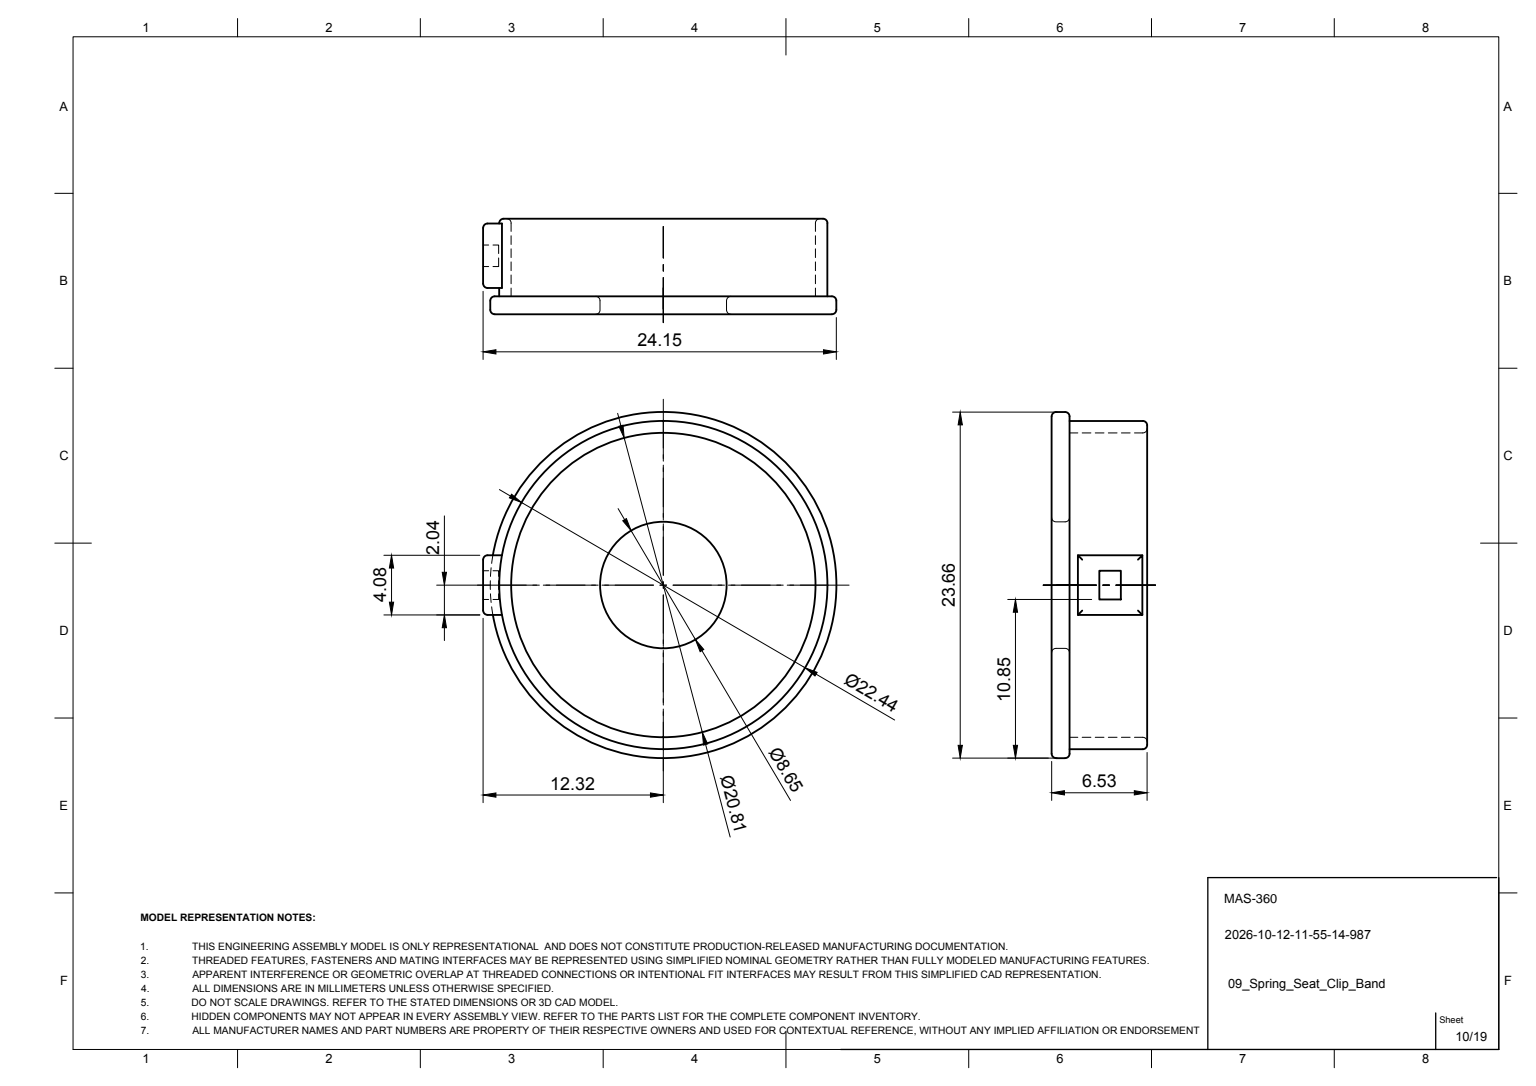
ISO-10303-21;
HEADER;
/* Generated by software containing ST-Developer
 * from STEP Tools, Inc. (www.steptools.com) 
 */

FILE_DESCRIPTION(
/* description */ (''),
/* implementation_level */ '2;1');

FILE_NAME(
/* name */ '09_Spring_Seat_Clip_Band.step',
/* time_stamp */ '2026-11-04T18:53:29-08:00',
/* author */ (''),
/* organization */ (''),
/* preprocessor_version */ 'ST-DEVELOPER v20.2',
/* originating_system */ 'Autodesk Translation Framework v15.17.0.0',
/* authorisation */ '');

FILE_SCHEMA (('AUTOMOTIVE_DESIGN { 1 0 10303 214 3 1 1 }'));
ENDSEC;

DATA;
#10=MECHANICAL_DESIGN_GEOMETRIC_PRESENTATION_REPRESENTATION('',(#1335),#100031);
#1007=CIRCLE('',#22159,4.6248);
#1008=CIRCLE('',#22160,0.3);
#1009=CIRCLE('',#22161,4.3248);
#1010=CIRCLE('',#22162,4.3248);
#1011=CIRCLE('',#22164,4.3248);
#1012=CIRCLE('',#22165,4.3248);
#1013=CIRCLE('',#22167,11.532);
#1014=CIRCLE('',#22169,0.3);
#1015=CIRCLE('',#22170,4.6248);
#1016=CIRCLE('',#22172,10.404);
#1017=CIRCLE('',#22174,10.404);
#1018=CIRCLE('',#22175,0.3);
#1019=CIRCLE('',#22176,10.704);
#1020=CIRCLE('',#22177,10.404);
#1021=CIRCLE('',#22179,10.92);
#1022=CIRCLE('',#22182,0.3);
#1023=CIRCLE('',#22183,11.22);
#1024=CIRCLE('',#22184,11.22);
#1025=CIRCLE('',#22186,11.22);
#1026=CIRCLE('',#22187,11.22);
#1027=CIRCLE('',#22188,11.22);
#1028=CIRCLE('',#22190,11.532);
#1029=CIRCLE('',#22191,0.3);
#1030=CIRCLE('',#22192,11.832);
#1031=CIRCLE('',#22193,11.832);
#1032=CIRCLE('',#22195,11.832);
#1033=CIRCLE('',#22196,11.832);
#1034=CIRCLE('',#22199,0.3);
#1276=TOROIDAL_SURFACE('',#22158,4.6248,0.3);
#1277=TOROIDAL_SURFACE('',#22168,4.6248,0.3);
#1278=TOROIDAL_SURFACE('',#22173,10.704,0.3);
#1279=TOROIDAL_SURFACE('',#22181,10.92,0.3);
#1280=TOROIDAL_SURFACE('',#22189,11.532,0.3);
#1281=TOROIDAL_SURFACE('',#22198,11.532,0.3);
#1299=SHAPE_REPRESENTATION_RELATIONSHIP('SRR','None',#100109,#1317);
#1317=ADVANCED_BREP_SHAPE_REPRESENTATION('',(#1353),#100021);
#1335=STYLED_ITEM('',(#100203),#1353);
#1353=MANIFOLD_SOLID_BREP('Body1',#20125);
#1638=PLANE('',#22166);
#1639=PLANE('',#22171);
#1640=PLANE('',#22178);
#1641=PLANE('',#22197);
#1642=PLANE('',#22208);
#1643=PLANE('',#22209);
#1644=PLANE('',#22210);
#1645=PLANE('',#22211);
#1646=PLANE('',#22212);
#1647=PLANE('',#22213);
#1648=PLANE('',#22214);
#1649=PLANE('',#22215);
#1650=PLANE('',#22216);
#1651=PLANE('',#22217);
#1776=FACE_BOUND('',#7253,.T.);
#1777=FACE_BOUND('',#7256,.T.);
#1778=FACE_BOUND('',#7259,.T.);
#1779=FACE_BOUND('',#7263,.T.);
#1780=FACE_BOUND('',#7267,.T.);
#1781=FACE_BOUND('',#7276,.T.);
#1974=ELLIPSE('',#22201,0.424264068711929,0.3);
#1975=ELLIPSE('',#22202,0.424264068711929,0.3);
#1976=ELLIPSE('',#22204,0.424264068711929,0.3);
#1977=ELLIPSE('',#22206,0.424264068711929,0.3);
#3153=LINE('',#97681,#4440);
#3154=LINE('',#97707,#4441);
#3155=LINE('',#97716,#4442);
#3156=LINE('',#97722,#4443);
#3157=LINE('',#97725,#4444);
#3158=LINE('',#97736,#4445);
#3159=LINE('',#97746,#4446);
#3160=LINE('',#97750,#4447);
#3161=LINE('',#97754,#4448);
#3162=LINE('',#97756,#4449);
#3163=LINE('',#97760,#4450);
#3164=LINE('',#97762,#4451);
#3165=LINE('',#97765,#4452);
#3166=LINE('',#97766,#4453);
#3167=LINE('',#97768,#4454);
#3168=LINE('',#97769,#4455);
#3169=LINE('',#97771,#4456);
#3170=LINE('',#97775,#4457);
#3171=LINE('',#97777,#4458);
#3172=LINE('',#97779,#4459);
#3173=LINE('',#97780,#4460);
#3174=LINE('',#97783,#4461);
#3175=LINE('',#97785,#4462);
#3176=LINE('',#97786,#4463);
#3177=LINE('',#97789,#4464);
#3178=LINE('',#97790,#4465);
#3179=LINE('',#97793,#4466);
#3180=LINE('',#97794,#4467);
#3181=LINE('',#97796,#4468);
#3182=LINE('',#97799,#4469);
#4440=VECTOR('',#27358,4.3248);
#4441=VECTOR('',#27393,10.404);
#4442=VECTOR('',#27404,11.22);
#4443=VECTOR('',#27409,10.);
#4444=VECTOR('',#27412,10.);
#4445=VECTOR('',#27425,11.832);
#4446=VECTOR('',#27438,10.);
#4447=VECTOR('',#27441,10.);
#4448=VECTOR('',#27446,10.);
#4449=VECTOR('',#27447,10.);
#4450=VECTOR('',#27452,10.);
#4451=VECTOR('',#27453,10.);
#4452=VECTOR('',#27458,10.);
#4453=VECTOR('',#27459,10.);
#4454=VECTOR('',#27462,10.);
#4455=VECTOR('',#27463,10.);
#4456=VECTOR('',#27466,10.);
#4457=VECTOR('',#27469,10.);
#4458=VECTOR('',#27470,10.);
#4459=VECTOR('',#27471,10.);
#4460=VECTOR('',#27472,10.);
#4461=VECTOR('',#27475,10.);
#4462=VECTOR('',#27476,10.);
#4463=VECTOR('',#27477,10.);
#4464=VECTOR('',#27480,10.);
#4465=VECTOR('',#27481,10.);
#4466=VECTOR('',#27484,10.);
#4467=VECTOR('',#27485,10.);
#4468=VECTOR('',#27488,10.);
#4469=VECTOR('',#27493,10.);
#4972=CYLINDRICAL_SURFACE('',#22163,4.3248);
#4973=CYLINDRICAL_SURFACE('',#22180,10.404);
#4974=CYLINDRICAL_SURFACE('',#22185,11.22);
#4975=CYLINDRICAL_SURFACE('',#22194,11.832);
#4976=CYLINDRICAL_SURFACE('',#22200,0.3);
#4977=CYLINDRICAL_SURFACE('',#22203,0.3);
#4978=CYLINDRICAL_SURFACE('',#22205,0.3);
#4979=CYLINDRICAL_SURFACE('',#22207,0.3);
#6011=FACE_OUTER_BOUND('',#7250,.T.);
#6012=FACE_OUTER_BOUND('',#7251,.T.);
#6013=FACE_OUTER_BOUND('',#7252,.T.);
#6014=FACE_OUTER_BOUND('',#7254,.T.);
#6015=FACE_OUTER_BOUND('',#7255,.T.);
#6016=FACE_OUTER_BOUND('',#7257,.T.);
#6017=FACE_OUTER_BOUND('',#7258,.T.);
#6018=FACE_OUTER_BOUND('',#7260,.T.);
#6019=FACE_OUTER_BOUND('',#7261,.T.);
#6020=FACE_OUTER_BOUND('',#7262,.T.);
#6021=FACE_OUTER_BOUND('',#7264,.T.);
#6022=FACE_OUTER_BOUND('',#7265,.T.);
#6023=FACE_OUTER_BOUND('',#7266,.T.);
#6024=FACE_OUTER_BOUND('',#7268,.T.);
#6025=FACE_OUTER_BOUND('',#7269,.T.);
#6026=FACE_OUTER_BOUND('',#7270,.T.);
#6027=FACE_OUTER_BOUND('',#7271,.T.);
#6028=FACE_OUTER_BOUND('',#7272,.T.);
#6029=FACE_OUTER_BOUND('',#7273,.T.);
#6030=FACE_OUTER_BOUND('',#7274,.T.);
#6031=FACE_OUTER_BOUND('',#7275,.T.);
#6032=FACE_OUTER_BOUND('',#7277,.T.);
#6033=FACE_OUTER_BOUND('',#7278,.T.);
#6034=FACE_OUTER_BOUND('',#7279,.T.);
#6035=FACE_OUTER_BOUND('',#7280,.T.);
#6036=FACE_OUTER_BOUND('',#7281,.T.);
#6037=FACE_OUTER_BOUND('',#7282,.T.);
#6038=FACE_OUTER_BOUND('',#7283,.T.);
#7250=EDGE_LOOP('',(#18177,#18178,#18179,#18180,#18181));
#7251=EDGE_LOOP('',(#18182,#18183,#18184,#18185,#18186,#18187));
#7252=EDGE_LOOP('',(#18188));
#7253=EDGE_LOOP('',(#18189));
#7254=EDGE_LOOP('',(#18190,#18191,#18192,#18193,#18194));
#7255=EDGE_LOOP('',(#18195));
#7256=EDGE_LOOP('',(#18196));
#7257=EDGE_LOOP('',(#18197,#18198,#18199,#18200,#18201));
#7258=EDGE_LOOP('',(#18202));
#7259=EDGE_LOOP('',(#18203));
#7260=EDGE_LOOP('',(#18204,#18205,#18206,#18207,#18208));
#7261=EDGE_LOOP('',(#18209,#18210,#18211,#18212,#18213));
#7262=EDGE_LOOP('',(#18214,#18215,#18216,#18217,#18218));
#7263=EDGE_LOOP('',(#18219,#18220,#18221,#18222));
#7264=EDGE_LOOP('',(#18223,#18224,#18225,#18226,#18227));
#7265=EDGE_LOOP('',(#18228,#18229,#18230,#18231,#18232,#18233));
#7266=EDGE_LOOP('',(#18234));
#7267=EDGE_LOOP('',(#18235));
#7268=EDGE_LOOP('',(#18236,#18237,#18238,#18239,#18240));
#7269=EDGE_LOOP('',(#18241,#18242,#18243,#18244));
#7270=EDGE_LOOP('',(#18245,#18246,#18247,#18248));
#7271=EDGE_LOOP('',(#18249,#18250,#18251,#18252));
#7272=EDGE_LOOP('',(#18253,#18254,#18255,#18256));
#7273=EDGE_LOOP('',(#18257,#18258,#18259,#18260));
#7274=EDGE_LOOP('',(#18261,#18262,#18263,#18264));
#7275=EDGE_LOOP('',(#18265,#18266,#18267,#18268));
#7276=EDGE_LOOP('',(#18269,#18270,#18271,#18272));
#7277=EDGE_LOOP('',(#18273,#18274,#18275,#18276));
#7278=EDGE_LOOP('',(#18277,#18278,#18279,#18280));
#7279=EDGE_LOOP('',(#18281,#18282,#18283,#18284));
#7280=EDGE_LOOP('',(#18285,#18286,#18287,#18288));
#7281=EDGE_LOOP('',(#18289,#18290,#18291,#18292));
#7282=EDGE_LOOP('',(#18293,#18294,#18295,#18296));
#7283=EDGE_LOOP('',(#18297,#18298,#18299,#18300));
#9719=VERTEX_POINT('',#97672);
#9720=VERTEX_POINT('',#97674);
#9721=VERTEX_POINT('',#97676);
#9722=VERTEX_POINT('',#97680);
#9723=VERTEX_POINT('',#97682);
#9724=VERTEX_POINT('',#97686);
#9725=VERTEX_POINT('',#97689);
#9726=VERTEX_POINT('',#97693);
#9727=VERTEX_POINT('',#97696);
#9728=VERTEX_POINT('',#97697);
#9729=VERTEX_POINT('',#97699);
#9730=VERTEX_POINT('',#97704);
#9731=VERTEX_POINT('',#97709);
#9732=VERTEX_POINT('',#97711);
#9733=VERTEX_POINT('',#97715);
#9734=VERTEX_POINT('',#97718);
#9735=VERTEX_POINT('',#97719);
#9736=VERTEX_POINT('',#97721);
#9737=VERTEX_POINT('',#97723);
#9738=VERTEX_POINT('',#97727);
#9739=VERTEX_POINT('',#97729);
#9740=VERTEX_POINT('',#97731);
#9741=VERTEX_POINT('',#97735);
#9742=VERTEX_POINT('',#97737);
#9743=VERTEX_POINT('',#97744);
#9744=VERTEX_POINT('',#97745);
#9745=VERTEX_POINT('',#97747);
#9746=VERTEX_POINT('',#97749);
#9747=VERTEX_POINT('',#97753);
#9748=VERTEX_POINT('',#97755);
#9749=VERTEX_POINT('',#97759);
#9750=VERTEX_POINT('',#97761);
#9751=VERTEX_POINT('',#97773);
#9752=VERTEX_POINT('',#97774);
#9753=VERTEX_POINT('',#97776);
#9754=VERTEX_POINT('',#97778);
#9755=VERTEX_POINT('',#97782);
#9756=VERTEX_POINT('',#97784);
#9757=VERTEX_POINT('',#97788);
#9758=VERTEX_POINT('',#97792);
#12563=EDGE_CURVE('',#9719,#9719,#1007,.T.);
#12564=EDGE_CURVE('',#9719,#9720,#1008,.T.);
#12565=EDGE_CURVE('',#9720,#9721,#1009,.T.);
#12566=EDGE_CURVE('',#9721,#9720,#1010,.T.);
#12567=EDGE_CURVE('',#9721,#9722,#3153,.T.);
#12568=EDGE_CURVE('',#9723,#9722,#1011,.T.);
#12569=EDGE_CURVE('',#9722,#9723,#1012,.T.);
#12570=EDGE_CURVE('',#9724,#9724,#1013,.T.);
#12571=EDGE_CURVE('',#9723,#9725,#1014,.T.);
#12572=EDGE_CURVE('',#9725,#9725,#1015,.T.);
#12573=EDGE_CURVE('',#9726,#9726,#1016,.T.);
#12574=EDGE_CURVE('',#9727,#9728,#1017,.T.);
#12575=EDGE_CURVE('',#9728,#9729,#1018,.T.);
#12576=EDGE_CURVE('',#9729,#9729,#1019,.T.);
#12577=EDGE_CURVE('',#9728,#9727,#1020,.T.);
#12578=EDGE_CURVE('',#9730,#9730,#1021,.T.);
#12579=EDGE_CURVE('',#9726,#9727,#3154,.T.);
#12580=EDGE_CURVE('',#9730,#9731,#1022,.T.);
#12581=EDGE_CURVE('',#9731,#9732,#1023,.T.);
#12582=EDGE_CURVE('',#9732,#9731,#1024,.T.);
#12583=EDGE_CURVE('',#9732,#9733,#3155,.T.);
#12584=EDGE_CURVE('',#9733,#9733,#1025,.T.);
#12585=EDGE_CURVE('',#9734,#9735,#1026,.T.);
#12586=EDGE_CURVE('',#9735,#9736,#3156,.T.);
#12587=EDGE_CURVE('',#9736,#9737,#1027,.T.);
#12588=EDGE_CURVE('',#9737,#9734,#3157,.T.);
#12589=EDGE_CURVE('',#9738,#9738,#1028,.T.);
#12590=EDGE_CURVE('',#9738,#9739,#1029,.T.);
#12591=EDGE_CURVE('',#9739,#9740,#1030,.T.);
#12592=EDGE_CURVE('',#9740,#9739,#1031,.T.);
#12593=EDGE_CURVE('',#9740,#9741,#3158,.T.);
#12594=EDGE_CURVE('',#9742,#9741,#1032,.T.);
#12595=EDGE_CURVE('',#9741,#9742,#1033,.T.);
#12596=EDGE_CURVE('',#9742,#9724,#1034,.T.);
#12597=EDGE_CURVE('',#9743,#9744,#3159,.T.);
#12598=EDGE_CURVE('',#9744,#9745,#1974,.T.);
#12599=EDGE_CURVE('',#9745,#9746,#3160,.T.);
#12600=EDGE_CURVE('',#9746,#9743,#1975,.T.);
#12601=EDGE_CURVE('',#9747,#9745,#3161,.T.);
#12602=EDGE_CURVE('',#9744,#9748,#3162,.T.);
#12603=EDGE_CURVE('',#9748,#9747,#1976,.T.);
#12604=EDGE_CURVE('',#9749,#9743,#3163,.T.);
#12605=EDGE_CURVE('',#9746,#9750,#3164,.T.);
#12606=EDGE_CURVE('',#9750,#9749,#1977,.T.);
#12607=EDGE_CURVE('',#9748,#9749,#3165,.T.);
#12608=EDGE_CURVE('',#9750,#9747,#3166,.T.);
#12609=EDGE_CURVE('',#9735,#9744,#3167,.T.);
#12610=EDGE_CURVE('',#9748,#9734,#3168,.T.);
#12611=EDGE_CURVE('',#9743,#9736,#3169,.T.);
#12612=EDGE_CURVE('',#9751,#9752,#3170,.T.);
#12613=EDGE_CURVE('',#9752,#9753,#3171,.T.);
#12614=EDGE_CURVE('',#9753,#9754,#3172,.T.);
#12615=EDGE_CURVE('',#9754,#9751,#3173,.T.);
#12616=EDGE_CURVE('',#9751,#9755,#3174,.T.);
#12617=EDGE_CURVE('',#9755,#9756,#3175,.T.);
#12618=EDGE_CURVE('',#9752,#9756,#3176,.T.);
#12619=EDGE_CURVE('',#9754,#9757,#3177,.T.);
#12620=EDGE_CURVE('',#9757,#9755,#3178,.T.);
#12621=EDGE_CURVE('',#9753,#9758,#3179,.T.);
#12622=EDGE_CURVE('',#9758,#9757,#3180,.T.);
#12623=EDGE_CURVE('',#9756,#9758,#3181,.T.);
#12624=EDGE_CURVE('',#9737,#9749,#3182,.T.);
#18177=ORIENTED_EDGE('',*,*,#12563,.T.);
#18178=ORIENTED_EDGE('',*,*,#12564,.T.);
#18179=ORIENTED_EDGE('',*,*,#12565,.T.);
#18180=ORIENTED_EDGE('',*,*,#12566,.T.);
#18181=ORIENTED_EDGE('',*,*,#12564,.F.);
#18182=ORIENTED_EDGE('',*,*,#12566,.F.);
#18183=ORIENTED_EDGE('',*,*,#12567,.T.);
#18184=ORIENTED_EDGE('',*,*,#12568,.F.);
#18185=ORIENTED_EDGE('',*,*,#12569,.F.);
#18186=ORIENTED_EDGE('',*,*,#12567,.F.);
#18187=ORIENTED_EDGE('',*,*,#12565,.F.);
#18188=ORIENTED_EDGE('',*,*,#12570,.F.);
#18189=ORIENTED_EDGE('',*,*,#12563,.F.);
#18190=ORIENTED_EDGE('',*,*,#12568,.T.);
#18191=ORIENTED_EDGE('',*,*,#12569,.T.);
#18192=ORIENTED_EDGE('',*,*,#12571,.T.);
#18193=ORIENTED_EDGE('',*,*,#12572,.T.);
#18194=ORIENTED_EDGE('',*,*,#12571,.F.);
#18195=ORIENTED_EDGE('',*,*,#12573,.T.);
#18196=ORIENTED_EDGE('',*,*,#12572,.F.);
#18197=ORIENTED_EDGE('',*,*,#12574,.T.);
#18198=ORIENTED_EDGE('',*,*,#12575,.T.);
#18199=ORIENTED_EDGE('',*,*,#12576,.T.);
#18200=ORIENTED_EDGE('',*,*,#12575,.F.);
#18201=ORIENTED_EDGE('',*,*,#12577,.T.);
#18202=ORIENTED_EDGE('',*,*,#12578,.F.);
#18203=ORIENTED_EDGE('',*,*,#12576,.F.);
#18204=ORIENTED_EDGE('',*,*,#12573,.F.);
#18205=ORIENTED_EDGE('',*,*,#12579,.T.);
#18206=ORIENTED_EDGE('',*,*,#12577,.F.);
#18207=ORIENTED_EDGE('',*,*,#12574,.F.);
#18208=ORIENTED_EDGE('',*,*,#12579,.F.);
#18209=ORIENTED_EDGE('',*,*,#12578,.T.);
#18210=ORIENTED_EDGE('',*,*,#12580,.T.);
#18211=ORIENTED_EDGE('',*,*,#12581,.T.);
#18212=ORIENTED_EDGE('',*,*,#12582,.T.);
#18213=ORIENTED_EDGE('',*,*,#12580,.F.);
#18214=ORIENTED_EDGE('',*,*,#12582,.F.);
#18215=ORIENTED_EDGE('',*,*,#12583,.T.);
#18216=ORIENTED_EDGE('',*,*,#12584,.T.);
#18217=ORIENTED_EDGE('',*,*,#12583,.F.);
#18218=ORIENTED_EDGE('',*,*,#12581,.F.);
#18219=ORIENTED_EDGE('',*,*,#12585,.T.);
#18220=ORIENTED_EDGE('',*,*,#12586,.T.);
#18221=ORIENTED_EDGE('',*,*,#12587,.T.);
#18222=ORIENTED_EDGE('',*,*,#12588,.T.);
#18223=ORIENTED_EDGE('',*,*,#12589,.T.);
#18224=ORIENTED_EDGE('',*,*,#12590,.T.);
#18225=ORIENTED_EDGE('',*,*,#12591,.T.);
#18226=ORIENTED_EDGE('',*,*,#12592,.T.);
#18227=ORIENTED_EDGE('',*,*,#12590,.F.);
#18228=ORIENTED_EDGE('',*,*,#12592,.F.);
#18229=ORIENTED_EDGE('',*,*,#12593,.T.);
#18230=ORIENTED_EDGE('',*,*,#12594,.F.);
#18231=ORIENTED_EDGE('',*,*,#12595,.F.);
#18232=ORIENTED_EDGE('',*,*,#12593,.F.);
#18233=ORIENTED_EDGE('',*,*,#12591,.F.);
#18234=ORIENTED_EDGE('',*,*,#12589,.F.);
#18235=ORIENTED_EDGE('',*,*,#12584,.F.);
#18236=ORIENTED_EDGE('',*,*,#12594,.T.);
#18237=ORIENTED_EDGE('',*,*,#12595,.T.);
#18238=ORIENTED_EDGE('',*,*,#12596,.T.);
#18239=ORIENTED_EDGE('',*,*,#12570,.T.);
#18240=ORIENTED_EDGE('',*,*,#12596,.F.);
#18241=ORIENTED_EDGE('',*,*,#12597,.T.);
#18242=ORIENTED_EDGE('',*,*,#12598,.T.);
#18243=ORIENTED_EDGE('',*,*,#12599,.T.);
#18244=ORIENTED_EDGE('',*,*,#12600,.T.);
#18245=ORIENTED_EDGE('',*,*,#12601,.T.);
#18246=ORIENTED_EDGE('',*,*,#12598,.F.);
#18247=ORIENTED_EDGE('',*,*,#12602,.T.);
#18248=ORIENTED_EDGE('',*,*,#12603,.T.);
#18249=ORIENTED_EDGE('',*,*,#12604,.T.);
#18250=ORIENTED_EDGE('',*,*,#12600,.F.);
#18251=ORIENTED_EDGE('',*,*,#12605,.T.);
#18252=ORIENTED_EDGE('',*,*,#12606,.T.);
#18253=ORIENTED_EDGE('',*,*,#12607,.T.);
#18254=ORIENTED_EDGE('',*,*,#12606,.F.);
#18255=ORIENTED_EDGE('',*,*,#12608,.T.);
#18256=ORIENTED_EDGE('',*,*,#12603,.F.);
#18257=ORIENTED_EDGE('',*,*,#12602,.F.);
#18258=ORIENTED_EDGE('',*,*,#12609,.F.);
#18259=ORIENTED_EDGE('',*,*,#12585,.F.);
#18260=ORIENTED_EDGE('',*,*,#12610,.F.);
#18261=ORIENTED_EDGE('',*,*,#12597,.F.);
#18262=ORIENTED_EDGE('',*,*,#12611,.T.);
#18263=ORIENTED_EDGE('',*,*,#12586,.F.);
#18264=ORIENTED_EDGE('',*,*,#12609,.T.);
#18265=ORIENTED_EDGE('',*,*,#12599,.F.);
#18266=ORIENTED_EDGE('',*,*,#12601,.F.);
#18267=ORIENTED_EDGE('',*,*,#12608,.F.);
#18268=ORIENTED_EDGE('',*,*,#12605,.F.);
#18269=ORIENTED_EDGE('',*,*,#12612,.T.);
#18270=ORIENTED_EDGE('',*,*,#12613,.T.);
#18271=ORIENTED_EDGE('',*,*,#12614,.T.);
#18272=ORIENTED_EDGE('',*,*,#12615,.T.);
#18273=ORIENTED_EDGE('',*,*,#12612,.F.);
#18274=ORIENTED_EDGE('',*,*,#12616,.T.);
#18275=ORIENTED_EDGE('',*,*,#12617,.T.);
#18276=ORIENTED_EDGE('',*,*,#12618,.F.);
#18277=ORIENTED_EDGE('',*,*,#12615,.F.);
#18278=ORIENTED_EDGE('',*,*,#12619,.T.);
#18279=ORIENTED_EDGE('',*,*,#12620,.T.);
#18280=ORIENTED_EDGE('',*,*,#12616,.F.);
#18281=ORIENTED_EDGE('',*,*,#12614,.F.);
#18282=ORIENTED_EDGE('',*,*,#12621,.T.);
#18283=ORIENTED_EDGE('',*,*,#12622,.T.);
#18284=ORIENTED_EDGE('',*,*,#12619,.F.);
#18285=ORIENTED_EDGE('',*,*,#12613,.F.);
#18286=ORIENTED_EDGE('',*,*,#12618,.T.);
#18287=ORIENTED_EDGE('',*,*,#12623,.T.);
#18288=ORIENTED_EDGE('',*,*,#12621,.F.);
#18289=ORIENTED_EDGE('',*,*,#12623,.F.);
#18290=ORIENTED_EDGE('',*,*,#12617,.F.);
#18291=ORIENTED_EDGE('',*,*,#12620,.F.);
#18292=ORIENTED_EDGE('',*,*,#12622,.F.);
#18293=ORIENTED_EDGE('',*,*,#12604,.F.);
#18294=ORIENTED_EDGE('',*,*,#12624,.F.);
#18295=ORIENTED_EDGE('',*,*,#12587,.F.);
#18296=ORIENTED_EDGE('',*,*,#12611,.F.);
#18297=ORIENTED_EDGE('',*,*,#12607,.F.);
#18298=ORIENTED_EDGE('',*,*,#12610,.T.);
#18299=ORIENTED_EDGE('',*,*,#12588,.F.);
#18300=ORIENTED_EDGE('',*,*,#12624,.T.);
#19945=ADVANCED_FACE('',(#6011),#1276,.T.);
#19946=ADVANCED_FACE('',(#6012),#4972,.F.);
#19947=ADVANCED_FACE('',(#6013,#1776),#1638,.T.);
#19948=ADVANCED_FACE('',(#6014),#1277,.T.);
#19949=ADVANCED_FACE('',(#6015,#1777),#1639,.T.);
#19950=ADVANCED_FACE('',(#6016),#1278,.T.);
#19951=ADVANCED_FACE('',(#6017,#1778),#1640,.T.);
#19952=ADVANCED_FACE('',(#6018),#4973,.F.);
#19953=ADVANCED_FACE('',(#6019),#1279,.T.);
#19954=ADVANCED_FACE('',(#6020,#1779),#4974,.T.);
#19955=ADVANCED_FACE('',(#6021),#1280,.T.);
#19956=ADVANCED_FACE('',(#6022),#4975,.T.);
#19957=ADVANCED_FACE('',(#6023,#1780),#1641,.T.);
#19958=ADVANCED_FACE('',(#6024),#1281,.T.);
#19959=ADVANCED_FACE('',(#6025),#4976,.T.);
#19960=ADVANCED_FACE('',(#6026),#4977,.T.);
#19961=ADVANCED_FACE('',(#6027),#4978,.T.);
#19962=ADVANCED_FACE('',(#6028),#4979,.T.);
#19963=ADVANCED_FACE('',(#6029),#1642,.T.);
#19964=ADVANCED_FACE('',(#6030),#1643,.F.);
#19965=ADVANCED_FACE('',(#6031,#1781),#1644,.T.);
#19966=ADVANCED_FACE('',(#6032),#1645,.F.);
#19967=ADVANCED_FACE('',(#6033),#1646,.F.);
#19968=ADVANCED_FACE('',(#6034),#1647,.F.);
#19969=ADVANCED_FACE('',(#6035),#1648,.F.);
#19970=ADVANCED_FACE('',(#6036),#1649,.F.);
#19971=ADVANCED_FACE('',(#6037),#1650,.T.);
#19972=ADVANCED_FACE('',(#6038),#1651,.T.);
#20125=CLOSED_SHELL('',(#19945,#19946,#19947,#19948,#19949,#19950,#19951,
#19952,#19953,#19954,#19955,#19956,#19957,#19958,#19959,#19960,#19961,#19962,
#19963,#19964,#19965,#19966,#19967,#19968,#19969,#19970,#19971,#19972));
#22157=AXIS2_PLACEMENT_3D('',#97670,#27344,#27345);
#22158=AXIS2_PLACEMENT_3D('',#97671,#27346,#27347);
#22159=AXIS2_PLACEMENT_3D('',#97673,#27348,#27349);
#22160=AXIS2_PLACEMENT_3D('',#97675,#27350,#27351);
#22161=AXIS2_PLACEMENT_3D('',#97677,#27352,#27353);
#22162=AXIS2_PLACEMENT_3D('',#97678,#27354,#27355);
#22163=AXIS2_PLACEMENT_3D('',#97679,#27356,#27357);
#22164=AXIS2_PLACEMENT_3D('',#97683,#27359,#27360);
#22165=AXIS2_PLACEMENT_3D('',#97684,#27361,#27362);
#22166=AXIS2_PLACEMENT_3D('',#97685,#27363,#27364);
#22167=AXIS2_PLACEMENT_3D('',#97687,#27365,#27366);
#22168=AXIS2_PLACEMENT_3D('',#97688,#27367,#27368);
#22169=AXIS2_PLACEMENT_3D('',#97690,#27369,#27370);
#22170=AXIS2_PLACEMENT_3D('',#97691,#27371,#27372);
#22171=AXIS2_PLACEMENT_3D('',#97692,#27373,#27374);
#22172=AXIS2_PLACEMENT_3D('',#97694,#27375,#27376);
#22173=AXIS2_PLACEMENT_3D('',#97695,#27377,#27378);
#22174=AXIS2_PLACEMENT_3D('',#97698,#27379,#27380);
#22175=AXIS2_PLACEMENT_3D('',#97700,#27381,#27382);
#22176=AXIS2_PLACEMENT_3D('',#97701,#27383,#27384);
#22177=AXIS2_PLACEMENT_3D('',#97702,#27385,#27386);
#22178=AXIS2_PLACEMENT_3D('',#97703,#27387,#27388);
#22179=AXIS2_PLACEMENT_3D('',#97705,#27389,#27390);
#22180=AXIS2_PLACEMENT_3D('',#97706,#27391,#27392);
#22181=AXIS2_PLACEMENT_3D('',#97708,#27394,#27395);
#22182=AXIS2_PLACEMENT_3D('',#97710,#27396,#27397);
#22183=AXIS2_PLACEMENT_3D('',#97712,#27398,#27399);
#22184=AXIS2_PLACEMENT_3D('',#97713,#27400,#27401);
#22185=AXIS2_PLACEMENT_3D('',#97714,#27402,#27403);
#22186=AXIS2_PLACEMENT_3D('',#97717,#27405,#27406);
#22187=AXIS2_PLACEMENT_3D('',#97720,#27407,#27408);
#22188=AXIS2_PLACEMENT_3D('',#97724,#27410,#27411);
#22189=AXIS2_PLACEMENT_3D('',#97726,#27413,#27414);
#22190=AXIS2_PLACEMENT_3D('',#97728,#27415,#27416);
#22191=AXIS2_PLACEMENT_3D('',#97730,#27417,#27418);
#22192=AXIS2_PLACEMENT_3D('',#97732,#27419,#27420);
#22193=AXIS2_PLACEMENT_3D('',#97733,#27421,#27422);
#22194=AXIS2_PLACEMENT_3D('',#97734,#27423,#27424);
#22195=AXIS2_PLACEMENT_3D('',#97738,#27426,#27427);
#22196=AXIS2_PLACEMENT_3D('',#97739,#27428,#27429);
#22197=AXIS2_PLACEMENT_3D('',#97740,#27430,#27431);
#22198=AXIS2_PLACEMENT_3D('',#97741,#27432,#27433);
#22199=AXIS2_PLACEMENT_3D('',#97742,#27434,#27435);
#22200=AXIS2_PLACEMENT_3D('',#97743,#27436,#27437);
#22201=AXIS2_PLACEMENT_3D('',#97748,#27439,#27440);
#22202=AXIS2_PLACEMENT_3D('',#97751,#27442,#27443);
#22203=AXIS2_PLACEMENT_3D('',#97752,#27444,#27445);
#22204=AXIS2_PLACEMENT_3D('',#97757,#27448,#27449);
#22205=AXIS2_PLACEMENT_3D('',#97758,#27450,#27451);
#22206=AXIS2_PLACEMENT_3D('',#97763,#27454,#27455);
#22207=AXIS2_PLACEMENT_3D('',#97764,#27456,#27457);
#22208=AXIS2_PLACEMENT_3D('',#97767,#27460,#27461);
#22209=AXIS2_PLACEMENT_3D('',#97770,#27464,#27465);
#22210=AXIS2_PLACEMENT_3D('',#97772,#27467,#27468);
#22211=AXIS2_PLACEMENT_3D('',#97781,#27473,#27474);
#22212=AXIS2_PLACEMENT_3D('',#97787,#27478,#27479);
#22213=AXIS2_PLACEMENT_3D('',#97791,#27482,#27483);
#22214=AXIS2_PLACEMENT_3D('',#97795,#27486,#27487);
#22215=AXIS2_PLACEMENT_3D('',#97797,#27489,#27490);
#22216=AXIS2_PLACEMENT_3D('',#97798,#27491,#27492);
#22217=AXIS2_PLACEMENT_3D('',#97800,#27494,#27495);
#27344=DIRECTION('axis',(0.,0.,1.));
#27345=DIRECTION('refdir',(1.,0.,0.));
#27346=DIRECTION('center_axis',(1.,0.,0.));
#27347=DIRECTION('ref_axis',(0.,0.,-1.));
#27348=DIRECTION('center_axis',(-1.,0.,0.));
#27349=DIRECTION('ref_axis',(0.,-1.,1.83697019872103E-16));
#27350=DIRECTION('center_axis',(0.,-1.,-1.22464679914735E-16));
#27351=DIRECTION('ref_axis',(0.,-1.22464679914735E-16,1.));
#27352=DIRECTION('center_axis',(1.,0.,0.));
#27353=DIRECTION('ref_axis',(0.,-1.,1.83697019872103E-16));
#27354=DIRECTION('center_axis',(1.,0.,0.));
#27355=DIRECTION('ref_axis',(0.,-1.,1.83697019872103E-16));
#27356=DIRECTION('center_axis',(1.,0.,0.));
#27357=DIRECTION('ref_axis',(0.,1.,0.));
#27358=DIRECTION('',(1.,0.,0.));
#27359=DIRECTION('center_axis',(-1.,0.,0.));
#27360=DIRECTION('ref_axis',(0.,-1.,1.83697019872103E-16));
#27361=DIRECTION('center_axis',(-1.,0.,0.));
#27362=DIRECTION('ref_axis',(0.,-1.,1.83697019872103E-16));
#27363=DIRECTION('center_axis',(-1.,0.,0.));
#27364=DIRECTION('ref_axis',(0.,0.,1.));
#27365=DIRECTION('center_axis',(1.,0.,0.));
#27366=DIRECTION('ref_axis',(0.,-1.,1.83697019872103E-16));
#27367=DIRECTION('center_axis',(1.,0.,0.));
#27368=DIRECTION('ref_axis',(0.,0.,-1.));
#27369=DIRECTION('center_axis',(0.,-1.,-1.22464679914735E-16));
#27370=DIRECTION('ref_axis',(0.,-1.22464679914735E-16,1.));
#27371=DIRECTION('center_axis',(1.,0.,0.));
#27372=DIRECTION('ref_axis',(0.,-1.,1.83697019872103E-16));
#27373=DIRECTION('center_axis',(1.,0.,0.));
#27374=DIRECTION('ref_axis',(0.,0.,-1.));
#27375=DIRECTION('center_axis',(1.,0.,0.));
#27376=DIRECTION('ref_axis',(0.,0.,-1.));
#27377=DIRECTION('center_axis',(1.,0.,0.));
#27378=DIRECTION('ref_axis',(0.,0.,-1.));
#27379=DIRECTION('center_axis',(-1.,0.,0.));
#27380=DIRECTION('ref_axis',(0.,-1.,1.83697019872103E-16));
#27381=DIRECTION('center_axis',(0.,-1.,-1.22464679914735E-16));
#27382=DIRECTION('ref_axis',(0.,-1.22464679914735E-16,1.));
#27383=DIRECTION('center_axis',(1.,0.,0.));
#27384=DIRECTION('ref_axis',(0.,-1.,1.83697019872103E-16));
#27385=DIRECTION('center_axis',(-1.,0.,0.));
#27386=DIRECTION('ref_axis',(0.,-1.,1.83697019872103E-16));
#27387=DIRECTION('center_axis',(1.,0.,0.));
#27388=DIRECTION('ref_axis',(0.,0.,-1.));
#27389=DIRECTION('center_axis',(-1.,0.,0.));
#27390=DIRECTION('ref_axis',(0.,-1.,1.83697019872103E-16));
#27391=DIRECTION('center_axis',(1.,0.,0.));
#27392=DIRECTION('ref_axis',(0.,1.,0.));
#27393=DIRECTION('',(1.,0.,0.));
#27394=DIRECTION('center_axis',(1.,0.,0.));
#27395=DIRECTION('ref_axis',(0.,0.,-1.));
#27396=DIRECTION('center_axis',(0.,-1.,-1.22464679914735E-16));
#27397=DIRECTION('ref_axis',(0.,-1.22464679914735E-16,1.));
#27398=DIRECTION('center_axis',(1.,0.,0.));
#27399=DIRECTION('ref_axis',(0.,-1.,1.83697019872103E-16));
#27400=DIRECTION('center_axis',(1.,0.,0.));
#27401=DIRECTION('ref_axis',(0.,-1.,1.83697019872103E-16));
#27402=DIRECTION('center_axis',(1.,0.,0.));
#27403=DIRECTION('ref_axis',(0.,1.,0.));
#27404=DIRECTION('',(-1.,0.,0.));
#27405=DIRECTION('center_axis',(1.,0.,0.));
#27406=DIRECTION('ref_axis',(0.,0.,-1.));
#27407=DIRECTION('center_axis',(1.,0.,0.));
#27408=DIRECTION('ref_axis',(0.,1.,0.));
#27409=DIRECTION('',(-1.,0.,0.));
#27410=DIRECTION('center_axis',(-1.,0.,0.));
#27411=DIRECTION('ref_axis',(0.,1.,0.));
#27412=DIRECTION('',(1.,0.,0.));
#27413=DIRECTION('center_axis',(1.,0.,0.));
#27414=DIRECTION('ref_axis',(0.,0.,-1.));
#27415=DIRECTION('center_axis',(-1.,0.,0.));
#27416=DIRECTION('ref_axis',(0.,-1.,1.83697019872103E-16));
#27417=DIRECTION('center_axis',(0.,-1.,-1.22464679914735E-16));
#27418=DIRECTION('ref_axis',(0.,-1.22464679914735E-16,1.));
#27419=DIRECTION('center_axis',(1.,0.,0.));
#27420=DIRECTION('ref_axis',(0.,-1.,1.83697019872103E-16));
#27421=DIRECTION('center_axis',(1.,0.,0.));
#27422=DIRECTION('ref_axis',(0.,-1.,1.83697019872103E-16));
#27423=DIRECTION('center_axis',(1.,0.,0.));
#27424=DIRECTION('ref_axis',(0.,1.,0.));
#27425=DIRECTION('',(-1.,0.,0.));
#27426=DIRECTION('center_axis',(-1.,0.,0.));
#27427=DIRECTION('ref_axis',(0.,-1.,1.83697019872103E-16));
#27428=DIRECTION('center_axis',(-1.,0.,0.));
#27429=DIRECTION('ref_axis',(0.,-1.,1.83697019872103E-16));
#27430=DIRECTION('center_axis',(1.,0.,0.));
#27431=DIRECTION('ref_axis',(0.,0.,-1.));
#27432=DIRECTION('center_axis',(1.,0.,0.));
#27433=DIRECTION('ref_axis',(0.,0.,-1.));
#27434=DIRECTION('center_axis',(0.,-1.,-1.22464679914735E-16));
#27435=DIRECTION('ref_axis',(0.,-1.22464679914735E-16,1.));
#27436=DIRECTION('center_axis',(-1.,0.,0.));
#27437=DIRECTION('ref_axis',(0.,-0.70710678118655,0.707106781186545));
#27438=DIRECTION('',(1.,0.,0.));
#27439=DIRECTION('center_axis',(-0.707106781186548,-0.707106781186548,0.));
#27440=DIRECTION('ref_axis',(0.707106781186547,-0.707106781186547,0.));
#27441=DIRECTION('',(-1.,0.,0.));
#27442=DIRECTION('center_axis',(0.707106781186548,-0.707106781186548,0.));
#27443=DIRECTION('ref_axis',(0.707106781186547,0.707106781186547,0.));
#27444=DIRECTION('center_axis',(0.,1.,0.));
#27445=DIRECTION('ref_axis',(0.707106781186545,0.,0.70710678118655));
#27446=DIRECTION('',(0.,-1.,0.));
#27447=DIRECTION('',(0.,1.,0.));
#27448=DIRECTION('center_axis',(0.707106781186548,-0.707106781186548,0.));
#27449=DIRECTION('ref_axis',(-0.707106781186547,-0.707106781186547,0.));
#27450=DIRECTION('center_axis',(0.,1.,0.));
#27451=DIRECTION('ref_axis',(-0.70710678118655,0.,0.707106781186545));
#27452=DIRECTION('',(0.,-1.,0.));
#27453=DIRECTION('',(0.,1.,0.));
#27454=DIRECTION('center_axis',(-0.707106781186548,-0.707106781186548,0.));
#27455=DIRECTION('ref_axis',(0.707106781186547,-0.707106781186547,0.));
#27456=DIRECTION('center_axis',(1.,0.,0.));
#27457=DIRECTION('ref_axis',(0.,0.70710678118655,0.707106781186545));
#27458=DIRECTION('',(-1.,0.,0.));
#27459=DIRECTION('',(1.,0.,0.));
#27460=DIRECTION('center_axis',(1.,0.,0.));
#27461=DIRECTION('ref_axis',(0.,0.,-1.));
#27462=DIRECTION('',(0.,0.,1.));
#27463=DIRECTION('',(0.,0.,-1.));
#27464=DIRECTION('center_axis',(0.,1.,0.));
#27465=DIRECTION('ref_axis',(1.,0.,0.));
#27466=DIRECTION('',(0.,0.,-1.));
#27467=DIRECTION('center_axis',(0.,0.,1.));
#27468=DIRECTION('ref_axis',(1.,0.,0.));
#27469=DIRECTION('',(-1.,0.,0.));
#27470=DIRECTION('',(0.,1.,0.));
#27471=DIRECTION('',(1.,0.,0.));
#27472=DIRECTION('',(0.,-1.,0.));
#27473=DIRECTION('center_axis',(0.,-1.,0.));
#27474=DIRECTION('ref_axis',(-1.,0.,0.));
#27475=DIRECTION('',(0.,0.,-1.));
#27476=DIRECTION('',(-1.,0.,0.));
#27477=DIRECTION('',(0.,0.,-1.));
#27478=DIRECTION('center_axis',(1.,0.,0.));
#27479=DIRECTION('ref_axis',(0.,-1.,0.));
#27480=DIRECTION('',(0.,0.,-1.));
#27481=DIRECTION('',(0.,-1.,0.));
#27482=DIRECTION('center_axis',(0.,1.,0.));
#27483=DIRECTION('ref_axis',(1.,0.,0.));
#27484=DIRECTION('',(0.,0.,-1.));
#27485=DIRECTION('',(1.,0.,0.));
#27486=DIRECTION('center_axis',(-1.,0.,0.));
#27487=DIRECTION('ref_axis',(0.,1.,0.));
#27488=DIRECTION('',(0.,1.,0.));
#27489=DIRECTION('center_axis',(0.,0.,-1.));
#27490=DIRECTION('ref_axis',(-1.,0.,0.));
#27491=DIRECTION('center_axis',(-1.,0.,0.));
#27492=DIRECTION('ref_axis',(0.,0.,1.));
#27493=DIRECTION('',(0.,0.,1.));
#27494=DIRECTION('center_axis',(0.,1.,0.));
#27495=DIRECTION('ref_axis',(0.,0.,1.));
#97670=CARTESIAN_POINT('',(0.,0.,0.));
#97671=CARTESIAN_POINT('Origin',(0.3,0.,0.));
#97672=CARTESIAN_POINT('',(0.,-5.66374651669668E-16,4.6248));
#97673=CARTESIAN_POINT('Origin',(0.,0.,0.));
#97674=CARTESIAN_POINT('',(0.3,-5.29635247695247E-16,4.3248));
#97675=CARTESIAN_POINT('Origin',(0.3,-5.66374651669668E-16,4.6248));
#97676=CARTESIAN_POINT('',(0.3,-4.3248,-5.29635247695247E-16));
#97677=CARTESIAN_POINT('Origin',(0.3,0.,0.));
#97678=CARTESIAN_POINT('Origin',(0.3,0.,0.));
#97679=CARTESIAN_POINT('Origin',(0.612,0.,0.));
#97680=CARTESIAN_POINT('',(0.924,-4.3248,-5.29635247695247E-16));
#97681=CARTESIAN_POINT('',(0.612,-4.3248,-5.29635247695247E-16));
#97682=CARTESIAN_POINT('',(0.924,-5.29635247695247E-16,4.3248));
#97683=CARTESIAN_POINT('Origin',(0.924,0.,0.));
#97684=CARTESIAN_POINT('Origin',(0.924,0.,0.));
#97685=CARTESIAN_POINT('Origin',(0.,11.832,0.));
#97686=CARTESIAN_POINT('',(0.,-1.41226268877673E-15,11.532));
#97687=CARTESIAN_POINT('Origin',(0.,0.,0.));
#97688=CARTESIAN_POINT('Origin',(0.924,0.,0.));
#97689=CARTESIAN_POINT('',(1.224,-5.66374651669668E-16,4.6248));
#97690=CARTESIAN_POINT('Origin',(0.924,-5.66374651669668E-16,4.6248));
#97691=CARTESIAN_POINT('Origin',(1.224,0.,0.));
#97692=CARTESIAN_POINT('Origin',(1.224,4.3248,0.));
#97693=CARTESIAN_POINT('',(1.224,-10.404,-1.27412252983291E-15));
#97694=CARTESIAN_POINT('Origin',(1.224,0.,0.));
#97695=CARTESIAN_POINT('Origin',(6.228,0.,0.));
#97696=CARTESIAN_POINT('',(6.228,-10.404,-1.27412252983291E-15));
#97697=CARTESIAN_POINT('',(6.228,-1.27412252983291E-15,10.404));
#97698=CARTESIAN_POINT('Origin',(6.228,0.,0.));
#97699=CARTESIAN_POINT('',(6.528,-1.31086193380733E-15,10.704));
#97700=CARTESIAN_POINT('Origin',(6.228,-1.31086193380733E-15,10.704));
#97701=CARTESIAN_POINT('Origin',(6.528,0.,0.));
#97702=CARTESIAN_POINT('Origin',(6.228,0.,0.));
#97703=CARTESIAN_POINT('Origin',(6.528,10.404,0.));
#97704=CARTESIAN_POINT('',(6.528,-1.33731430466891E-15,10.92));
#97705=CARTESIAN_POINT('Origin',(6.528,0.,0.));
#97706=CARTESIAN_POINT('Origin',(3.876,0.,0.));
#97707=CARTESIAN_POINT('',(3.876,-10.404,-1.27412252983291E-15));
#97708=CARTESIAN_POINT('Origin',(6.228,0.,0.));
#97709=CARTESIAN_POINT('',(6.228,-1.37405370864333E-15,11.22));
#97710=CARTESIAN_POINT('Origin',(6.228,-1.33731430466891E-15,10.92));
#97711=CARTESIAN_POINT('',(6.228,-11.22,-1.37405370864333E-15));
#97712=CARTESIAN_POINT('Origin',(6.228,0.,0.));
#97713=CARTESIAN_POINT('Origin',(6.228,0.,0.));
#97714=CARTESIAN_POINT('Origin',(3.876,0.,0.));
#97715=CARTESIAN_POINT('',(1.224,-11.22,-1.37405370864333E-15));
#97716=CARTESIAN_POINT('',(3.876,-11.22,-1.37405370864333E-15));
#97717=CARTESIAN_POINT('Origin',(1.224,0.,0.));
#97718=CARTESIAN_POINT('',(6.2016,2.04,11.0329869029198));
#97719=CARTESIAN_POINT('',(6.2016,-2.04,11.0329869029198));
#97720=CARTESIAN_POINT('Origin',(6.2016,0.,0.));
#97721=CARTESIAN_POINT('',(1.7952,-2.04,11.0329869029198));
#97722=CARTESIAN_POINT('',(3.876,-2.04,11.0329869029198));
#97723=CARTESIAN_POINT('',(1.7952,2.04,11.0329869029198));
#97724=CARTESIAN_POINT('Origin',(1.7952,0.,0.));
#97725=CARTESIAN_POINT('',(3.876,2.04,11.0329869029198));
#97726=CARTESIAN_POINT('Origin',(0.924,0.,0.));
#97727=CARTESIAN_POINT('',(1.224,-1.41226268877673E-15,11.532));
#97728=CARTESIAN_POINT('Origin',(1.224,0.,0.));
#97729=CARTESIAN_POINT('',(0.924,-1.44900209275115E-15,11.832));
#97730=CARTESIAN_POINT('Origin',(0.924,-1.41226268877673E-15,11.532));
#97731=CARTESIAN_POINT('',(0.924,-11.832,-1.44900209275115E-15));
#97732=CARTESIAN_POINT('Origin',(0.924,0.,0.));
#97733=CARTESIAN_POINT('Origin',(0.924,0.,0.));
#97734=CARTESIAN_POINT('Origin',(0.612,0.,0.));
#97735=CARTESIAN_POINT('',(0.3,-11.832,-1.44900209275115E-15));
#97736=CARTESIAN_POINT('',(0.612,-11.832,-1.44900209275115E-15));
#97737=CARTESIAN_POINT('',(0.3,-1.44900209275115E-15,11.832));
#97738=CARTESIAN_POINT('Origin',(0.3,0.,0.));
#97739=CARTESIAN_POINT('Origin',(0.3,0.,0.));
#97740=CARTESIAN_POINT('Origin',(1.224,11.22,0.));
#97741=CARTESIAN_POINT('Origin',(0.3,0.,0.));
#97742=CARTESIAN_POINT('Origin',(0.3,-1.41226268877673E-15,11.532));
#97743=CARTESIAN_POINT('Origin',(2.8968,-1.74,12.0216));
#97744=CARTESIAN_POINT('',(1.7952,-2.04,12.0216));
#97745=CARTESIAN_POINT('',(6.2016,-2.04,12.0216));
#97746=CARTESIAN_POINT('',(2.8968,-2.04,12.0216));
#97747=CARTESIAN_POINT('',(5.9016,-1.74,12.3216));
#97748=CARTESIAN_POINT('Origin',(5.9016,-1.74,12.0216));
#97749=CARTESIAN_POINT('',(2.0952,-1.74,12.3216));
#97750=CARTESIAN_POINT('',(2.8968,-1.74,12.3216));
#97751=CARTESIAN_POINT('Origin',(2.0952,-1.74,12.0216));
#97752=CARTESIAN_POINT('Origin',(5.9016,-2.04,12.0216));
#97753=CARTESIAN_POINT('',(5.9016,1.74,12.3216));
#97754=CARTESIAN_POINT('',(5.9016,-2.04,12.3216));
#97755=CARTESIAN_POINT('',(6.2016,2.04,12.0216));
#97756=CARTESIAN_POINT('',(6.2016,-2.04,12.0216));
#97757=CARTESIAN_POINT('Origin',(5.9016,1.74,12.0216));
#97758=CARTESIAN_POINT('Origin',(2.0952,-2.04,12.0216));
#97759=CARTESIAN_POINT('',(1.7952,2.04,12.0216));
#97760=CARTESIAN_POINT('',(1.7952,-2.04,12.0216));
#97761=CARTESIAN_POINT('',(2.0952,1.74,12.3216));
#97762=CARTESIAN_POINT('',(2.0952,-2.04,12.3216));
#97763=CARTESIAN_POINT('Origin',(2.0952,1.74,12.0216));
#97764=CARTESIAN_POINT('Origin',(2.8968,1.74,12.0216));
#97765=CARTESIAN_POINT('',(2.8968,2.04,12.0216));
#97766=CARTESIAN_POINT('',(2.8968,1.74,12.3216));
#97767=CARTESIAN_POINT('Origin',(6.2016,-2.04,12.3216));
#97768=CARTESIAN_POINT('',(6.2016,-2.04,10.8528));
#97769=CARTESIAN_POINT('',(6.2016,2.04,10.8528));
#97770=CARTESIAN_POINT('Origin',(3.9984,-2.04,11.5872));
#97771=CARTESIAN_POINT('',(1.7952,-2.04,12.3216));
#97772=CARTESIAN_POINT('Origin',(1.7952,-2.04,12.3216));
#97773=CARTESIAN_POINT('',(4.7328,-0.9792,12.3216));
#97774=CARTESIAN_POINT('',(3.264,-0.9792,12.3216));
#97775=CARTESIAN_POINT('',(3.264,-0.9792,12.3216));
#97776=CARTESIAN_POINT('',(3.264,0.9792,12.3216));
#97777=CARTESIAN_POINT('',(3.264,-1.5096,12.3216));
#97778=CARTESIAN_POINT('',(4.7328,0.9792,12.3216));
#97779=CARTESIAN_POINT('',(2.5296,0.9792,12.3216));
#97780=CARTESIAN_POINT('',(4.7328,-0.5304,12.3216));
#97781=CARTESIAN_POINT('Origin',(4.7328,-0.9792,12.3216));
#97782=CARTESIAN_POINT('',(4.7328,-0.9792,11.2608));
#97783=CARTESIAN_POINT('',(4.7328,-0.9792,12.3216));
#97784=CARTESIAN_POINT('',(3.264,-0.9792,11.2608));
#97785=CARTESIAN_POINT('',(3.264,-0.9792,11.2608));
#97786=CARTESIAN_POINT('',(3.264,-0.9792,12.3216));
#97787=CARTESIAN_POINT('Origin',(4.7328,0.9792,12.3216));
#97788=CARTESIAN_POINT('',(4.7328,0.9792,11.2608));
#97789=CARTESIAN_POINT('',(4.7328,0.9792,12.3216));
#97790=CARTESIAN_POINT('',(4.7328,-0.9792,11.2608));
#97791=CARTESIAN_POINT('Origin',(3.264,0.9792,12.3216));
#97792=CARTESIAN_POINT('',(3.264,0.9792,11.2608));
#97793=CARTESIAN_POINT('',(3.264,0.9792,12.3216));
#97794=CARTESIAN_POINT('',(4.7328,0.9792,11.2608));
#97795=CARTESIAN_POINT('Origin',(3.264,-0.9792,12.3216));
#97796=CARTESIAN_POINT('',(3.264,0.9792,11.2608));
#97797=CARTESIAN_POINT('Origin',(3.9984,0.,11.2608));
#97798=CARTESIAN_POINT('Origin',(1.7952,-2.04,10.8528));
#97799=CARTESIAN_POINT('',(1.7952,2.04,12.3216));
#97800=CARTESIAN_POINT('Origin',(3.9984,2.04,11.5872));
#100001=UNCERTAINTY_MEASURE_WITH_UNIT(LENGTH_MEASURE(0.01),#100032,
'DISTANCE_ACCURACY_VALUE',
'Maximum model space distance between geometric entities at asserted c
onnectivities');
#100011=UNCERTAINTY_MEASURE_WITH_UNIT(LENGTH_MEASURE(0.01),#100032,
'DISTANCE_ACCURACY_VALUE',
'Maximum model space distance between geometric entities at asserted c
onnectivities');
#100021=(
GEOMETRIC_REPRESENTATION_CONTEXT(3)
GLOBAL_UNCERTAINTY_ASSIGNED_CONTEXT((#100001))
GLOBAL_UNIT_ASSIGNED_CONTEXT((#100032,#100034,#100035))
REPRESENTATION_CONTEXT('','3D')
);
#100031=(
GEOMETRIC_REPRESENTATION_CONTEXT(3)
GLOBAL_UNCERTAINTY_ASSIGNED_CONTEXT((#100011))
GLOBAL_UNIT_ASSIGNED_CONTEXT((#100032,#100034,#100035))
REPRESENTATION_CONTEXT('','3D')
);
#100032=(
LENGTH_UNIT()
NAMED_UNIT(*)
SI_UNIT(.MILLI.,.METRE.)
);
#100034=(
NAMED_UNIT(*)
PLANE_ANGLE_UNIT()
SI_UNIT($,.RADIAN.)
);
#100035=(
NAMED_UNIT(*)
SI_UNIT($,.STERADIAN.)
SOLID_ANGLE_UNIT()
);
#100045=SHAPE_DEFINITION_REPRESENTATION(#100064,#100109);
#100064=PRODUCT_DEFINITION_SHAPE('',$,#100129);
#100109=SHAPE_REPRESENTATION('',(#22157),#100021);
#100119=PRODUCT_DEFINITION_CONTEXT('part definition',#100178,'design');
#100129=PRODUCT_DEFINITION('2026-10-12-11-55-14-987',
'09_Spring_Seat_Clip_Band',#100148,#100119);
#100148=PRODUCT_DEFINITION_FORMATION('',$,#100189);
#100178=APPLICATION_CONTEXT(
'Core Data for Automotive Mechanical Design Process');
#100179=PRODUCT_CONTEXT('part definition',#100178,'mechanical');
#100189=PRODUCT('2026-10-12-11-55-14-987','09_Spring_Seat_Clip_Band',$,
(#100179));
#100203=PRESENTATION_STYLE_ASSIGNMENT((#100209));
#100209=SURFACE_STYLE_USAGE(.BOTH.,#100215);
#100215=SURFACE_SIDE_STYLE('',(#100221));
#100221=SURFACE_STYLE_FILL_AREA(#100227);
#100227=FILL_AREA_STYLE('Opaque(122,133,145)',(#100233));
#100233=FILL_AREA_STYLE_COLOUR('Opaque(122,133,145)',#100239);
#100239=COLOUR_RGB('Opaque(122,133,145)',0.47843137254902,0.52156862745098,
0.568627450980392);
ENDSEC;
END-ISO-10303-21;
